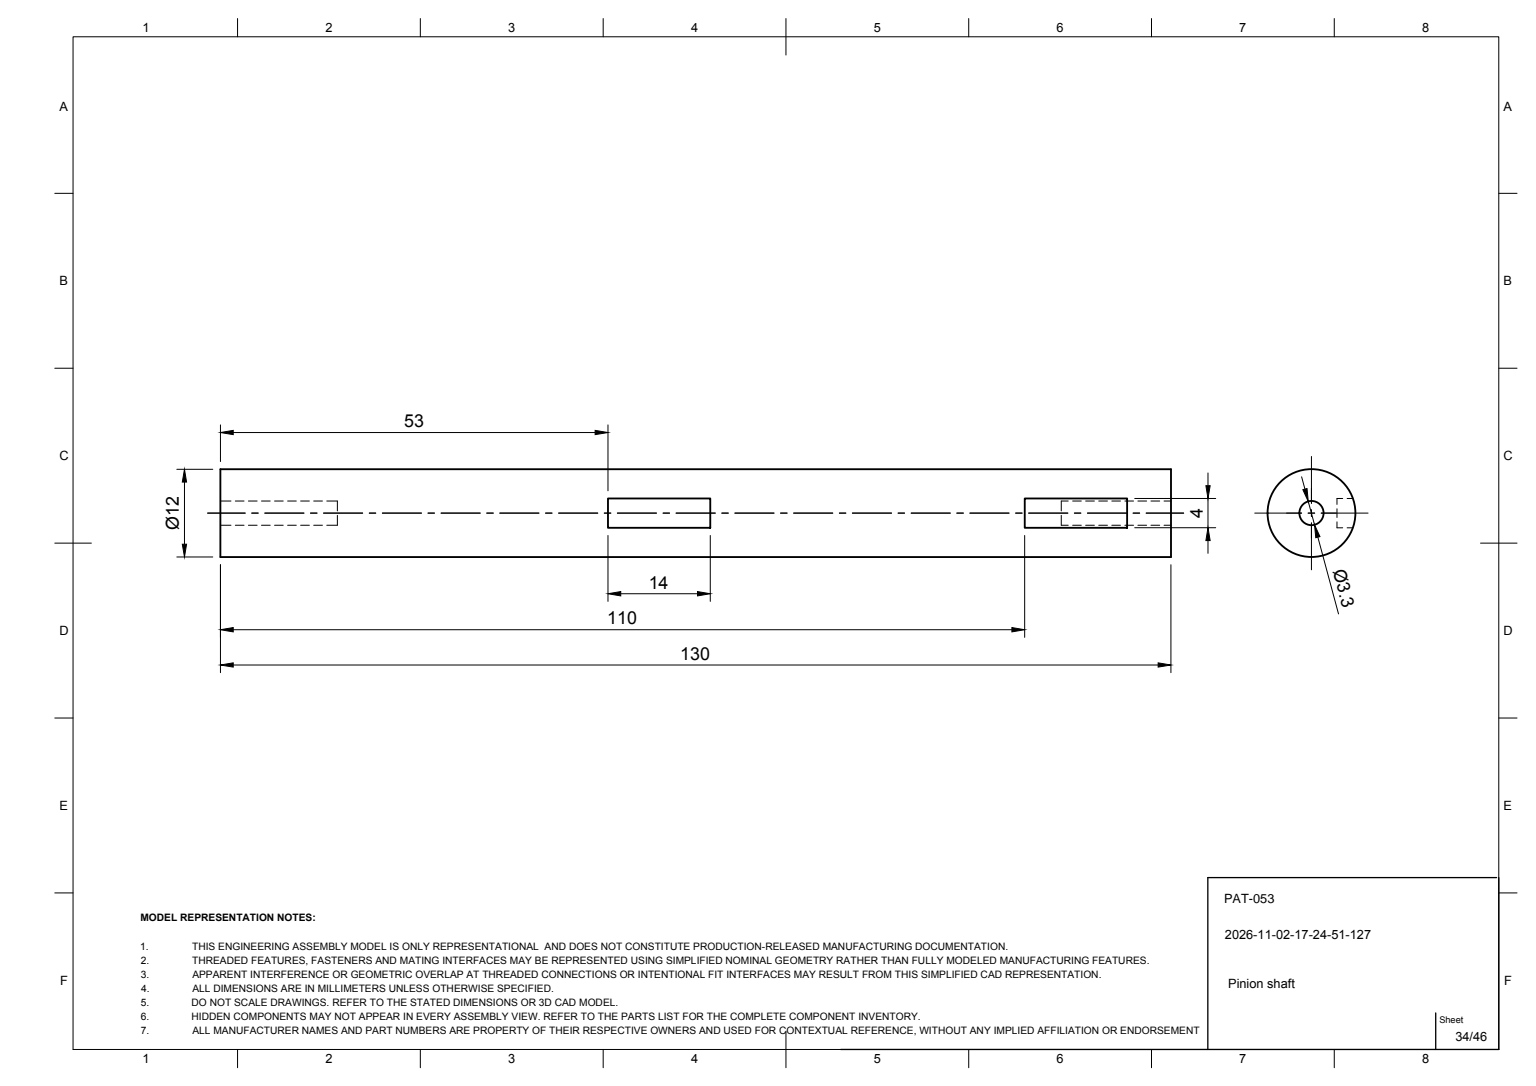
ISO-10303-21;
HEADER;
/* Generated by software containing ST-Developer
 * from STEP Tools, Inc. (www.steptools.com) 
 */

FILE_DESCRIPTION(
/* description */ ('Hand-operated arbor press'),
/* implementation_level */ '2;1');

FILE_NAME(
/* name */ 'Pinion shaft.step',
/* time_stamp */ '2026-10-28T03:25:25-07:00',
/* author */ (''),
/* organization */ (''),
/* preprocessor_version */ 'ST-DEVELOPER v20.2',
/* originating_system */ 'Autodesk Translation Framework v15.17.0.0',
/* authorisation */ '');

FILE_SCHEMA (('AUTOMOTIVE_DESIGN { 1 0 10303 214 3 1 1 }'));
ENDSEC;

DATA;
#10=MECHANICAL_DESIGN_GEOMETRIC_PRESENTATION_REPRESENTATION('',(#619),#32751);
#528=SHAPE_REPRESENTATION_RELATIONSHIP('SRR','None',#32960,#570);
#570=ADVANCED_BREP_SHAPE_REPRESENTATION('',(#666),#32734);
#619=STYLED_ITEM('',(#33242),#666);
#666=MANIFOLD_SOLID_BREP('Body1',#12518);
#817=FACE_BOUND('',#2607,.T.);
#818=FACE_BOUND('',#2608,.T.);
#819=FACE_BOUND('',#2610,.T.);
#820=FACE_BOUND('',#2612,.T.);
#1192=PLANE('',#13798);
#1193=PLANE('',#13802);
#1194=PLANE('',#13803);
#1195=PLANE('',#13804);
#1196=PLANE('',#13806);
#1197=PLANE('',#13807);
#1198=PLANE('',#13808);
#1199=PLANE('',#13810);
#1200=PLANE('',#13811);
#1201=PLANE('',#13813);
#1202=PLANE('',#13814);
#1203=PLANE('',#13815);
#1204=PLANE('',#13820);
#1205=PLANE('',#13821);
#1774=FACE_OUTER_BOUND('',#2592,.T.);
#1775=FACE_OUTER_BOUND('',#2593,.T.);
#1776=FACE_OUTER_BOUND('',#2594,.T.);
#1777=FACE_OUTER_BOUND('',#2595,.T.);
#1778=FACE_OUTER_BOUND('',#2596,.T.);
#1779=FACE_OUTER_BOUND('',#2597,.T.);
#1780=FACE_OUTER_BOUND('',#2598,.T.);
#1781=FACE_OUTER_BOUND('',#2599,.T.);
#1782=FACE_OUTER_BOUND('',#2600,.T.);
#1783=FACE_OUTER_BOUND('',#2601,.T.);
#1784=FACE_OUTER_BOUND('',#2602,.T.);
#1785=FACE_OUTER_BOUND('',#2603,.T.);
#1786=FACE_OUTER_BOUND('',#2604,.T.);
#1787=FACE_OUTER_BOUND('',#2605,.T.);
#1788=FACE_OUTER_BOUND('',#2606,.T.);
#1789=FACE_OUTER_BOUND('',#2609,.T.);
#1790=FACE_OUTER_BOUND('',#2611,.T.);
#2592=EDGE_LOOP('',(#10722,#10723,#10724,#10725));
#2593=EDGE_LOOP('',(#10726));
#2594=EDGE_LOOP('',(#10727,#10728,#10729,#10730));
#2595=EDGE_LOOP('',(#10731));
#2596=EDGE_LOOP('',(#10732,#10733,#10734,#10735));
#2597=EDGE_LOOP('',(#10736,#10737,#10738,#10739));
#2598=EDGE_LOOP('',(#10740,#10741,#10742,#10743));
#2599=EDGE_LOOP('',(#10744,#10745,#10746,#10747));
#2600=EDGE_LOOP('',(#10748,#10749,#10750,#10751));
#2601=EDGE_LOOP('',(#10752,#10753,#10754,#10755));
#2602=EDGE_LOOP('',(#10756,#10757,#10758,#10759));
#2603=EDGE_LOOP('',(#10760,#10761,#10762,#10763));
#2604=EDGE_LOOP('',(#10764,#10765,#10766,#10767));
#2605=EDGE_LOOP('',(#10768,#10769,#10770,#10771));
#2606=EDGE_LOOP('',(#10772,#10773,#10774,#10775));
#2607=EDGE_LOOP('',(#10776,#10777,#10778,#10779));
#2608=EDGE_LOOP('',(#10780,#10781,#10782,#10783));
#2609=EDGE_LOOP('',(#10784));
#2610=EDGE_LOOP('',(#10785));
#2611=EDGE_LOOP('',(#10786));
#2612=EDGE_LOOP('',(#10787));
#3731=LINE('',#20530,#4902);
#3732=LINE('',#20537,#4903);
#3733=LINE('',#20543,#4904);
#3734=LINE('',#20545,#4905);
#3735=LINE('',#20547,#4906);
#3736=LINE('',#20548,#4907);
#3737=LINE('',#20553,#4908);
#3738=LINE('',#20554,#4909);
#3739=LINE('',#20557,#4910);
#3740=LINE('',#20558,#4911);
#3741=LINE('',#20561,#4912);
#3742=LINE('',#20562,#4913);
#3743=LINE('',#20568,#4914);
#3744=LINE('',#20570,#4915);
#3745=LINE('',#20572,#4916);
#3746=LINE('',#20573,#4917);
#3747=LINE('',#20578,#4918);
#3748=LINE('',#20579,#4919);
#3749=LINE('',#20582,#4920);
#3750=LINE('',#20583,#4921);
#3751=LINE('',#20586,#4922);
#3752=LINE('',#20587,#4923);
#3753=LINE('',#20594,#4924);
#4902=VECTOR('',#16658,0.165);
#4903=VECTOR('',#16667,0.165);
#4904=VECTOR('',#16674,1.);
#4905=VECTOR('',#16675,1.);
#4906=VECTOR('',#16676,1.);
#4907=VECTOR('',#16677,1.);
#4908=VECTOR('',#16682,1.);
#4909=VECTOR('',#16683,1.);
#4910=VECTOR('',#16686,1.);
#4911=VECTOR('',#16687,1.);
#4912=VECTOR('',#16690,1.);
#4913=VECTOR('',#16691,1.);
#4914=VECTOR('',#16698,1.);
#4915=VECTOR('',#16699,1.);
#4916=VECTOR('',#16700,1.);
#4917=VECTOR('',#16701,1.);
#4918=VECTOR('',#16706,1.);
#4919=VECTOR('',#16707,1.);
#4920=VECTOR('',#16710,1.);
#4921=VECTOR('',#16711,1.);
#4922=VECTOR('',#16714,1.);
#4923=VECTOR('',#16715,1.);
#4924=VECTOR('',#16724,0.6);
#5440=CIRCLE('',#13796,0.165);
#5441=CIRCLE('',#13797,0.165);
#5442=CIRCLE('',#13800,0.165);
#5443=CIRCLE('',#13801,0.165);
#5444=CIRCLE('',#13805,0.6);
#5445=CIRCLE('',#13809,0.6);
#5446=CIRCLE('',#13812,0.6);
#5447=CIRCLE('',#13816,0.6);
#5448=CIRCLE('',#13818,0.6);
#5449=CIRCLE('',#13819,0.6);
#6361=VERTEX_POINT('',#20527);
#6362=VERTEX_POINT('',#20529);
#6363=VERTEX_POINT('',#20534);
#6364=VERTEX_POINT('',#20536);
#6365=VERTEX_POINT('',#20541);
#6366=VERTEX_POINT('',#20542);
#6367=VERTEX_POINT('',#20544);
#6368=VERTEX_POINT('',#20546);
#6369=VERTEX_POINT('',#20550);
#6370=VERTEX_POINT('',#20552);
#6371=VERTEX_POINT('',#20556);
#6372=VERTEX_POINT('',#20560);
#6373=VERTEX_POINT('',#20566);
#6374=VERTEX_POINT('',#20567);
#6375=VERTEX_POINT('',#20569);
#6376=VERTEX_POINT('',#20571);
#6377=VERTEX_POINT('',#20575);
#6378=VERTEX_POINT('',#20577);
#6379=VERTEX_POINT('',#20581);
#6380=VERTEX_POINT('',#20585);
#6381=VERTEX_POINT('',#20591);
#6382=VERTEX_POINT('',#20593);
#7864=EDGE_CURVE('',#6361,#6361,#5440,.T.);
#7865=EDGE_CURVE('',#6361,#6362,#3731,.T.);
#7866=EDGE_CURVE('',#6362,#6362,#5441,.T.);
#7867=EDGE_CURVE('',#6363,#6363,#5442,.T.);
#7868=EDGE_CURVE('',#6363,#6364,#3732,.T.);
#7869=EDGE_CURVE('',#6364,#6364,#5443,.T.);
#7870=EDGE_CURVE('',#6365,#6366,#3733,.T.);
#7871=EDGE_CURVE('',#6365,#6367,#3734,.T.);
#7872=EDGE_CURVE('',#6368,#6367,#3735,.T.);
#7873=EDGE_CURVE('',#6368,#6366,#3736,.T.);
#7874=EDGE_CURVE('',#6366,#6369,#5444,.T.);
#7875=EDGE_CURVE('',#6370,#6368,#3737,.T.);
#7876=EDGE_CURVE('',#6369,#6370,#3738,.T.);
#7877=EDGE_CURVE('',#6367,#6371,#3739,.T.);
#7878=EDGE_CURVE('',#6370,#6371,#3740,.T.);
#7879=EDGE_CURVE('',#6369,#6372,#3741,.T.);
#7880=EDGE_CURVE('',#6371,#6372,#3742,.T.);
#7881=EDGE_CURVE('',#6372,#6365,#5445,.T.);
#7882=EDGE_CURVE('',#6373,#6374,#3743,.T.);
#7883=EDGE_CURVE('',#6373,#6375,#3744,.T.);
#7884=EDGE_CURVE('',#6376,#6375,#3745,.T.);
#7885=EDGE_CURVE('',#6376,#6374,#3746,.T.);
#7886=EDGE_CURVE('',#6374,#6377,#5446,.T.);
#7887=EDGE_CURVE('',#6378,#6376,#3747,.T.);
#7888=EDGE_CURVE('',#6377,#6378,#3748,.T.);
#7889=EDGE_CURVE('',#6375,#6379,#3749,.T.);
#7890=EDGE_CURVE('',#6378,#6379,#3750,.T.);
#7891=EDGE_CURVE('',#6377,#6380,#3751,.T.);
#7892=EDGE_CURVE('',#6379,#6380,#3752,.T.);
#7893=EDGE_CURVE('',#6380,#6373,#5447,.T.);
#7894=EDGE_CURVE('',#6381,#6381,#5448,.T.);
#7895=EDGE_CURVE('',#6381,#6382,#3753,.T.);
#7896=EDGE_CURVE('',#6382,#6382,#5449,.T.);
#10722=ORIENTED_EDGE('',*,*,#7864,.F.);
#10723=ORIENTED_EDGE('',*,*,#7865,.T.);
#10724=ORIENTED_EDGE('',*,*,#7866,.F.);
#10725=ORIENTED_EDGE('',*,*,#7865,.F.);
#10726=ORIENTED_EDGE('',*,*,#7864,.T.);
#10727=ORIENTED_EDGE('',*,*,#7867,.F.);
#10728=ORIENTED_EDGE('',*,*,#7868,.T.);
#10729=ORIENTED_EDGE('',*,*,#7869,.T.);
#10730=ORIENTED_EDGE('',*,*,#7868,.F.);
#10731=ORIENTED_EDGE('',*,*,#7869,.F.);
#10732=ORIENTED_EDGE('',*,*,#7870,.F.);
#10733=ORIENTED_EDGE('',*,*,#7871,.T.);
#10734=ORIENTED_EDGE('',*,*,#7872,.F.);
#10735=ORIENTED_EDGE('',*,*,#7873,.T.);
#10736=ORIENTED_EDGE('',*,*,#7874,.F.);
#10737=ORIENTED_EDGE('',*,*,#7873,.F.);
#10738=ORIENTED_EDGE('',*,*,#7875,.F.);
#10739=ORIENTED_EDGE('',*,*,#7876,.F.);
#10740=ORIENTED_EDGE('',*,*,#7875,.T.);
#10741=ORIENTED_EDGE('',*,*,#7872,.T.);
#10742=ORIENTED_EDGE('',*,*,#7877,.T.);
#10743=ORIENTED_EDGE('',*,*,#7878,.F.);
#10744=ORIENTED_EDGE('',*,*,#7879,.F.);
#10745=ORIENTED_EDGE('',*,*,#7876,.T.);
#10746=ORIENTED_EDGE('',*,*,#7878,.T.);
#10747=ORIENTED_EDGE('',*,*,#7880,.T.);
#10748=ORIENTED_EDGE('',*,*,#7881,.F.);
#10749=ORIENTED_EDGE('',*,*,#7880,.F.);
#10750=ORIENTED_EDGE('',*,*,#7877,.F.);
#10751=ORIENTED_EDGE('',*,*,#7871,.F.);
#10752=ORIENTED_EDGE('',*,*,#7882,.F.);
#10753=ORIENTED_EDGE('',*,*,#7883,.T.);
#10754=ORIENTED_EDGE('',*,*,#7884,.F.);
#10755=ORIENTED_EDGE('',*,*,#7885,.T.);
#10756=ORIENTED_EDGE('',*,*,#7886,.F.);
#10757=ORIENTED_EDGE('',*,*,#7885,.F.);
#10758=ORIENTED_EDGE('',*,*,#7887,.F.);
#10759=ORIENTED_EDGE('',*,*,#7888,.F.);
#10760=ORIENTED_EDGE('',*,*,#7887,.T.);
#10761=ORIENTED_EDGE('',*,*,#7884,.T.);
#10762=ORIENTED_EDGE('',*,*,#7889,.T.);
#10763=ORIENTED_EDGE('',*,*,#7890,.F.);
#10764=ORIENTED_EDGE('',*,*,#7891,.F.);
#10765=ORIENTED_EDGE('',*,*,#7888,.T.);
#10766=ORIENTED_EDGE('',*,*,#7890,.T.);
#10767=ORIENTED_EDGE('',*,*,#7892,.T.);
#10768=ORIENTED_EDGE('',*,*,#7893,.F.);
#10769=ORIENTED_EDGE('',*,*,#7892,.F.);
#10770=ORIENTED_EDGE('',*,*,#7889,.F.);
#10771=ORIENTED_EDGE('',*,*,#7883,.F.);
#10772=ORIENTED_EDGE('',*,*,#7894,.F.);
#10773=ORIENTED_EDGE('',*,*,#7895,.T.);
#10774=ORIENTED_EDGE('',*,*,#7896,.T.);
#10775=ORIENTED_EDGE('',*,*,#7895,.F.);
#10776=ORIENTED_EDGE('',*,*,#7879,.T.);
#10777=ORIENTED_EDGE('',*,*,#7881,.T.);
#10778=ORIENTED_EDGE('',*,*,#7870,.T.);
#10779=ORIENTED_EDGE('',*,*,#7874,.T.);
#10780=ORIENTED_EDGE('',*,*,#7891,.T.);
#10781=ORIENTED_EDGE('',*,*,#7893,.T.);
#10782=ORIENTED_EDGE('',*,*,#7882,.T.);
#10783=ORIENTED_EDGE('',*,*,#7886,.T.);
#10784=ORIENTED_EDGE('',*,*,#7894,.T.);
#10785=ORIENTED_EDGE('',*,*,#7866,.T.);
#10786=ORIENTED_EDGE('',*,*,#7896,.F.);
#10787=ORIENTED_EDGE('',*,*,#7867,.T.);
#11751=CYLINDRICAL_SURFACE('',#13795,0.165);
#11752=CYLINDRICAL_SURFACE('',#13799,0.165);
#11753=CYLINDRICAL_SURFACE('',#13817,0.6);
#12283=ADVANCED_FACE('',(#1774),#11751,.F.);
#12284=ADVANCED_FACE('',(#1775),#1192,.T.);
#12285=ADVANCED_FACE('',(#1776),#11752,.F.);
#12286=ADVANCED_FACE('',(#1777),#1193,.F.);
#12287=ADVANCED_FACE('',(#1778),#1194,.F.);
#12288=ADVANCED_FACE('',(#1779),#1195,.T.);
#12289=ADVANCED_FACE('',(#1780),#1196,.F.);
#12290=ADVANCED_FACE('',(#1781),#1197,.F.);
#12291=ADVANCED_FACE('',(#1782),#1198,.F.);
#12292=ADVANCED_FACE('',(#1783),#1199,.F.);
#12293=ADVANCED_FACE('',(#1784),#1200,.T.);
#12294=ADVANCED_FACE('',(#1785),#1201,.F.);
#12295=ADVANCED_FACE('',(#1786),#1202,.F.);
#12296=ADVANCED_FACE('',(#1787),#1203,.F.);
#12297=ADVANCED_FACE('',(#1788,#817,#818),#11753,.T.);
#12298=ADVANCED_FACE('',(#1789,#819),#1204,.T.);
#12299=ADVANCED_FACE('',(#1790,#820),#1205,.F.);
#12518=CLOSED_SHELL('',(#12283,#12284,#12285,#12286,#12287,#12288,#12289,
#12290,#12291,#12292,#12293,#12294,#12295,#12296,#12297,#12298,#12299));
#13794=AXIS2_PLACEMENT_3D('',#20525,#16652,#16653);
#13795=AXIS2_PLACEMENT_3D('',#20526,#16654,#16655);
#13796=AXIS2_PLACEMENT_3D('',#20528,#16656,#16657);
#13797=AXIS2_PLACEMENT_3D('',#20531,#16659,#16660);
#13798=AXIS2_PLACEMENT_3D('',#20532,#16661,#16662);
#13799=AXIS2_PLACEMENT_3D('',#20533,#16663,#16664);
#13800=AXIS2_PLACEMENT_3D('',#20535,#16665,#16666);
#13801=AXIS2_PLACEMENT_3D('',#20538,#16668,#16669);
#13802=AXIS2_PLACEMENT_3D('',#20539,#16670,#16671);
#13803=AXIS2_PLACEMENT_3D('',#20540,#16672,#16673);
#13804=AXIS2_PLACEMENT_3D('',#20549,#16678,#16679);
#13805=AXIS2_PLACEMENT_3D('',#20551,#16680,#16681);
#13806=AXIS2_PLACEMENT_3D('',#20555,#16684,#16685);
#13807=AXIS2_PLACEMENT_3D('',#20559,#16688,#16689);
#13808=AXIS2_PLACEMENT_3D('',#20563,#16692,#16693);
#13809=AXIS2_PLACEMENT_3D('',#20564,#16694,#16695);
#13810=AXIS2_PLACEMENT_3D('',#20565,#16696,#16697);
#13811=AXIS2_PLACEMENT_3D('',#20574,#16702,#16703);
#13812=AXIS2_PLACEMENT_3D('',#20576,#16704,#16705);
#13813=AXIS2_PLACEMENT_3D('',#20580,#16708,#16709);
#13814=AXIS2_PLACEMENT_3D('',#20584,#16712,#16713);
#13815=AXIS2_PLACEMENT_3D('',#20588,#16716,#16717);
#13816=AXIS2_PLACEMENT_3D('',#20589,#16718,#16719);
#13817=AXIS2_PLACEMENT_3D('',#20590,#16720,#16721);
#13818=AXIS2_PLACEMENT_3D('',#20592,#16722,#16723);
#13819=AXIS2_PLACEMENT_3D('',#20595,#16725,#16726);
#13820=AXIS2_PLACEMENT_3D('',#20596,#16727,#16728);
#13821=AXIS2_PLACEMENT_3D('',#20597,#16729,#16730);
#16652=DIRECTION('axis',(0.,0.,1.));
#16653=DIRECTION('refdir',(1.,0.,0.));
#16654=DIRECTION('center_axis',(0.,1.,0.));
#16655=DIRECTION('ref_axis',(1.,0.,0.));
#16656=DIRECTION('center_axis',(0.,1.,0.));
#16657=DIRECTION('ref_axis',(1.,0.,0.));
#16658=DIRECTION('',(0.,1.,0.));
#16659=DIRECTION('center_axis',(0.,-1.,0.));
#16660=DIRECTION('ref_axis',(1.,0.,0.));
#16661=DIRECTION('center_axis',(0.,1.,0.));
#16662=DIRECTION('ref_axis',(1.,0.,0.));
#16663=DIRECTION('center_axis',(0.,1.,0.));
#16664=DIRECTION('ref_axis',(1.,0.,0.));
#16665=DIRECTION('center_axis',(0.,1.,0.));
#16666=DIRECTION('ref_axis',(1.,0.,0.));
#16667=DIRECTION('',(0.,1.,0.));
#16668=DIRECTION('center_axis',(0.,1.,0.));
#16669=DIRECTION('ref_axis',(1.,0.,0.));
#16670=DIRECTION('center_axis',(0.,1.,0.));
#16671=DIRECTION('ref_axis',(1.,0.,0.));
#16672=DIRECTION('center_axis',(0.,0.,-1.));
#16673=DIRECTION('ref_axis',(-1.,0.,0.));
#16674=DIRECTION('',(0.,-1.,0.));
#16675=DIRECTION('',(-1.,0.,0.));
#16676=DIRECTION('',(0.,1.,0.));
#16677=DIRECTION('',(1.,0.,0.));
#16678=DIRECTION('center_axis',(0.,1.,0.));
#16679=DIRECTION('ref_axis',(1.,0.,0.));
#16680=DIRECTION('center_axis',(0.,-1.,0.));
#16681=DIRECTION('ref_axis',(1.,0.,0.));
#16682=DIRECTION('',(0.,0.,-1.));
#16683=DIRECTION('',(-1.,0.,0.));
#16684=DIRECTION('center_axis',(-1.,0.,0.));
#16685=DIRECTION('ref_axis',(0.,0.,1.));
#16686=DIRECTION('',(0.,0.,1.));
#16687=DIRECTION('',(0.,1.,0.));
#16688=DIRECTION('center_axis',(0.,0.,1.));
#16689=DIRECTION('ref_axis',(1.,0.,0.));
#16690=DIRECTION('',(0.,1.,0.));
#16691=DIRECTION('',(1.,0.,0.));
#16692=DIRECTION('center_axis',(0.,1.,0.));
#16693=DIRECTION('ref_axis',(0.,0.,1.));
#16694=DIRECTION('center_axis',(0.,1.,0.));
#16695=DIRECTION('ref_axis',(1.,0.,0.));
#16696=DIRECTION('center_axis',(0.,0.,-1.));
#16697=DIRECTION('ref_axis',(-1.,0.,0.));
#16698=DIRECTION('',(0.,-1.,0.));
#16699=DIRECTION('',(-1.,0.,0.));
#16700=DIRECTION('',(0.,1.,0.));
#16701=DIRECTION('',(1.,0.,0.));
#16702=DIRECTION('center_axis',(0.,1.,0.));
#16703=DIRECTION('ref_axis',(1.,0.,0.));
#16704=DIRECTION('center_axis',(0.,-1.,0.));
#16705=DIRECTION('ref_axis',(1.,0.,0.));
#16706=DIRECTION('',(0.,0.,-1.));
#16707=DIRECTION('',(-1.,0.,0.));
#16708=DIRECTION('center_axis',(-1.,0.,0.));
#16709=DIRECTION('ref_axis',(0.,0.,1.));
#16710=DIRECTION('',(0.,0.,1.));
#16711=DIRECTION('',(0.,1.,0.));
#16712=DIRECTION('center_axis',(0.,0.,1.));
#16713=DIRECTION('ref_axis',(1.,0.,0.));
#16714=DIRECTION('',(0.,1.,0.));
#16715=DIRECTION('',(1.,0.,0.));
#16716=DIRECTION('center_axis',(0.,1.,0.));
#16717=DIRECTION('ref_axis',(0.,0.,1.));
#16718=DIRECTION('center_axis',(0.,1.,0.));
#16719=DIRECTION('ref_axis',(1.,0.,0.));
#16720=DIRECTION('center_axis',(0.,1.,0.));
#16721=DIRECTION('ref_axis',(1.,0.,0.));
#16722=DIRECTION('center_axis',(0.,1.,0.));
#16723=DIRECTION('ref_axis',(1.,0.,0.));
#16724=DIRECTION('',(0.,-1.,0.));
#16725=DIRECTION('center_axis',(0.,1.,0.));
#16726=DIRECTION('ref_axis',(1.,0.,0.));
#16727=DIRECTION('center_axis',(0.,1.,0.));
#16728=DIRECTION('ref_axis',(1.,0.,0.));
#16729=DIRECTION('center_axis',(0.,1.,0.));
#16730=DIRECTION('ref_axis',(1.,0.,0.));
#20525=CARTESIAN_POINT('',(0.,0.,0.));
#20526=CARTESIAN_POINT('Origin',(-3.25,6.,20.));
#20527=CARTESIAN_POINT('',(-3.415,6.,20.));
#20528=CARTESIAN_POINT('Origin',(-3.25,6.,20.));
#20529=CARTESIAN_POINT('',(-3.415,7.5,20.));
#20530=CARTESIAN_POINT('',(-3.415,6.,20.));
#20531=CARTESIAN_POINT('Origin',(-3.25,7.5,20.));
#20532=CARTESIAN_POINT('Origin',(-3.25,6.,20.));
#20533=CARTESIAN_POINT('Origin',(-3.25,-5.6,20.));
#20534=CARTESIAN_POINT('',(-3.415,-5.5,20.));
#20535=CARTESIAN_POINT('Origin',(-3.25,-5.5,20.));
#20536=CARTESIAN_POINT('',(-3.415,-3.9,20.));
#20537=CARTESIAN_POINT('',(-3.415,-5.6,20.));
#20538=CARTESIAN_POINT('Origin',(-3.25,-3.9,20.));
#20539=CARTESIAN_POINT('Origin',(-3.25,-3.9,20.));
#20540=CARTESIAN_POINT('Origin',(-2.55,5.5,19.8));
#20541=CARTESIAN_POINT('',(-2.68431457505076,6.9,19.8));
#20542=CARTESIAN_POINT('',(-2.68431457505076,5.5,19.8));
#20543=CARTESIAN_POINT('',(-2.68431457505076,-5.5,19.8));
#20544=CARTESIAN_POINT('',(-2.9,6.9,19.8));
#20545=CARTESIAN_POINT('',(-2.9,6.9,19.8));
#20546=CARTESIAN_POINT('',(-2.9,5.5,19.8));
#20547=CARTESIAN_POINT('',(-2.9,5.5,19.8));
#20548=CARTESIAN_POINT('',(-2.9,5.5,19.8));
#20549=CARTESIAN_POINT('Origin',(-2.725,5.5,20.));
#20550=CARTESIAN_POINT('',(-2.68431457505076,5.5,20.2));
#20551=CARTESIAN_POINT('Origin',(-3.25,5.5,20.));
#20552=CARTESIAN_POINT('',(-2.9,5.5,20.2));
#20553=CARTESIAN_POINT('',(-2.9,5.5,20.2));
#20554=CARTESIAN_POINT('',(-2.55,5.5,20.2));
#20555=CARTESIAN_POINT('Origin',(-2.9,5.5,19.8));
#20556=CARTESIAN_POINT('',(-2.9,6.9,20.2));
#20557=CARTESIAN_POINT('',(-2.9,6.9,20.2));
#20558=CARTESIAN_POINT('',(-2.9,5.5,20.2));
#20559=CARTESIAN_POINT('Origin',(-2.9,5.5,20.2));
#20560=CARTESIAN_POINT('',(-2.68431457505076,6.9,20.2));
#20561=CARTESIAN_POINT('',(-2.68431457505076,-5.5,20.2));
#20562=CARTESIAN_POINT('',(-2.55,6.9,20.2));
#20563=CARTESIAN_POINT('Origin',(-2.725,6.9,20.));
#20564=CARTESIAN_POINT('Origin',(-3.25,6.9,20.));
#20565=CARTESIAN_POINT('Origin',(-2.55,-0.2,19.8));
#20566=CARTESIAN_POINT('',(-2.68431457505076,1.2,19.8));
#20567=CARTESIAN_POINT('',(-2.68431457505076,-0.2,19.8));
#20568=CARTESIAN_POINT('',(-2.68431457505076,-5.5,19.8));
#20569=CARTESIAN_POINT('',(-2.9,1.2,19.8));
#20570=CARTESIAN_POINT('',(-2.9,1.2,19.8));
#20571=CARTESIAN_POINT('',(-2.9,-0.2,19.8));
#20572=CARTESIAN_POINT('',(-2.9,-0.2,19.8));
#20573=CARTESIAN_POINT('',(-2.9,-0.2,19.8));
#20574=CARTESIAN_POINT('Origin',(-2.725,-0.2,20.));
#20575=CARTESIAN_POINT('',(-2.68431457505076,-0.2,20.2));
#20576=CARTESIAN_POINT('Origin',(-3.25,-0.2,20.));
#20577=CARTESIAN_POINT('',(-2.9,-0.2,20.2));
#20578=CARTESIAN_POINT('',(-2.9,-0.2,20.2));
#20579=CARTESIAN_POINT('',(-2.55,-0.2,20.2));
#20580=CARTESIAN_POINT('Origin',(-2.9,-0.2,19.8));
#20581=CARTESIAN_POINT('',(-2.9,1.2,20.2));
#20582=CARTESIAN_POINT('',(-2.9,1.2,20.2));
#20583=CARTESIAN_POINT('',(-2.9,-0.2,20.2));
#20584=CARTESIAN_POINT('Origin',(-2.9,-0.2,20.2));
#20585=CARTESIAN_POINT('',(-2.68431457505076,1.2,20.2));
#20586=CARTESIAN_POINT('',(-2.68431457505076,-5.5,20.2));
#20587=CARTESIAN_POINT('',(-2.55,1.2,20.2));
#20588=CARTESIAN_POINT('Origin',(-2.725,1.2,20.));
#20589=CARTESIAN_POINT('Origin',(-3.25,1.2,20.));
#20590=CARTESIAN_POINT('Origin',(-3.25,-5.5,20.));
#20591=CARTESIAN_POINT('',(-3.85,7.5,20.));
#20592=CARTESIAN_POINT('Origin',(-3.25,7.5,20.));
#20593=CARTESIAN_POINT('',(-3.85,-5.5,20.));
#20594=CARTESIAN_POINT('',(-3.85,-5.5,20.));
#20595=CARTESIAN_POINT('Origin',(-3.25,-5.5,20.));
#20596=CARTESIAN_POINT('Origin',(-3.25,7.5,20.));
#20597=CARTESIAN_POINT('Origin',(-3.25,-5.5,20.));
#32685=UNCERTAINTY_MEASURE_WITH_UNIT(LENGTH_MEASURE(0.001),#32752,
'DISTANCE_ACCURACY_VALUE',
'Maximum model space distance between geometric entities at asserted c
onnectivities');
#32702=UNCERTAINTY_MEASURE_WITH_UNIT(LENGTH_MEASURE(0.001),#32752,
'DISTANCE_ACCURACY_VALUE',
'Maximum model space distance between geometric entities at asserted c
onnectivities');
#32734=(
GEOMETRIC_REPRESENTATION_CONTEXT(3)
GLOBAL_UNCERTAINTY_ASSIGNED_CONTEXT((#32685))
GLOBAL_UNIT_ASSIGNED_CONTEXT((#32752,#32754,#32755))
REPRESENTATION_CONTEXT('','3D')
);
#32751=(
GEOMETRIC_REPRESENTATION_CONTEXT(3)
GLOBAL_UNCERTAINTY_ASSIGNED_CONTEXT((#32702))
GLOBAL_UNIT_ASSIGNED_CONTEXT((#32752,#32754,#32755))
REPRESENTATION_CONTEXT('','3D')
);
#32752=(
LENGTH_UNIT()
NAMED_UNIT(*)
SI_UNIT(.CENTI.,.METRE.)
);
#32754=(
NAMED_UNIT(*)
PLANE_ANGLE_UNIT()
SI_UNIT($,.RADIAN.)
);
#32755=(
NAMED_UNIT(*)
SI_UNIT($,.STERADIAN.)
SOLID_ANGLE_UNIT()
);
#32787=SHAPE_DEFINITION_REPRESENTATION(#32844,#32960);
#32844=PRODUCT_DEFINITION_SHAPE('',$,#33009);
#32960=SHAPE_REPRESENTATION('',(#13794),#32734);
#32977=PRODUCT_DEFINITION_CONTEXT('part definition',#33123,'design');
#33009=PRODUCT_DEFINITION('Pinion shaft','Pinion shaft',#33057,#32977);
#33057=PRODUCT_DEFINITION_FORMATION('',$,#33156);
#33123=APPLICATION_CONTEXT(
'Core Data for Automotive Mechanical Design Process');
#33124=PRODUCT_CONTEXT('part definition',#33123,'mechanical');
#33156=PRODUCT('Pinion shaft','Pinion shaft','Pinion shaft',(#33124));
#33236=COLOUR_RGB('Grey',0.48,0.52,0.57);
#33237=FILL_AREA_STYLE_COLOUR('',#33236);
#33238=FILL_AREA_STYLE('',(#33237));
#33239=SURFACE_STYLE_FILL_AREA(#33238);
#33240=SURFACE_SIDE_STYLE('',(#33239));
#33241=SURFACE_STYLE_USAGE(.BOTH.,#33240);
#33242=PRESENTATION_STYLE_ASSIGNMENT((#33241));
ENDSEC;
END-ISO-10303-21;
